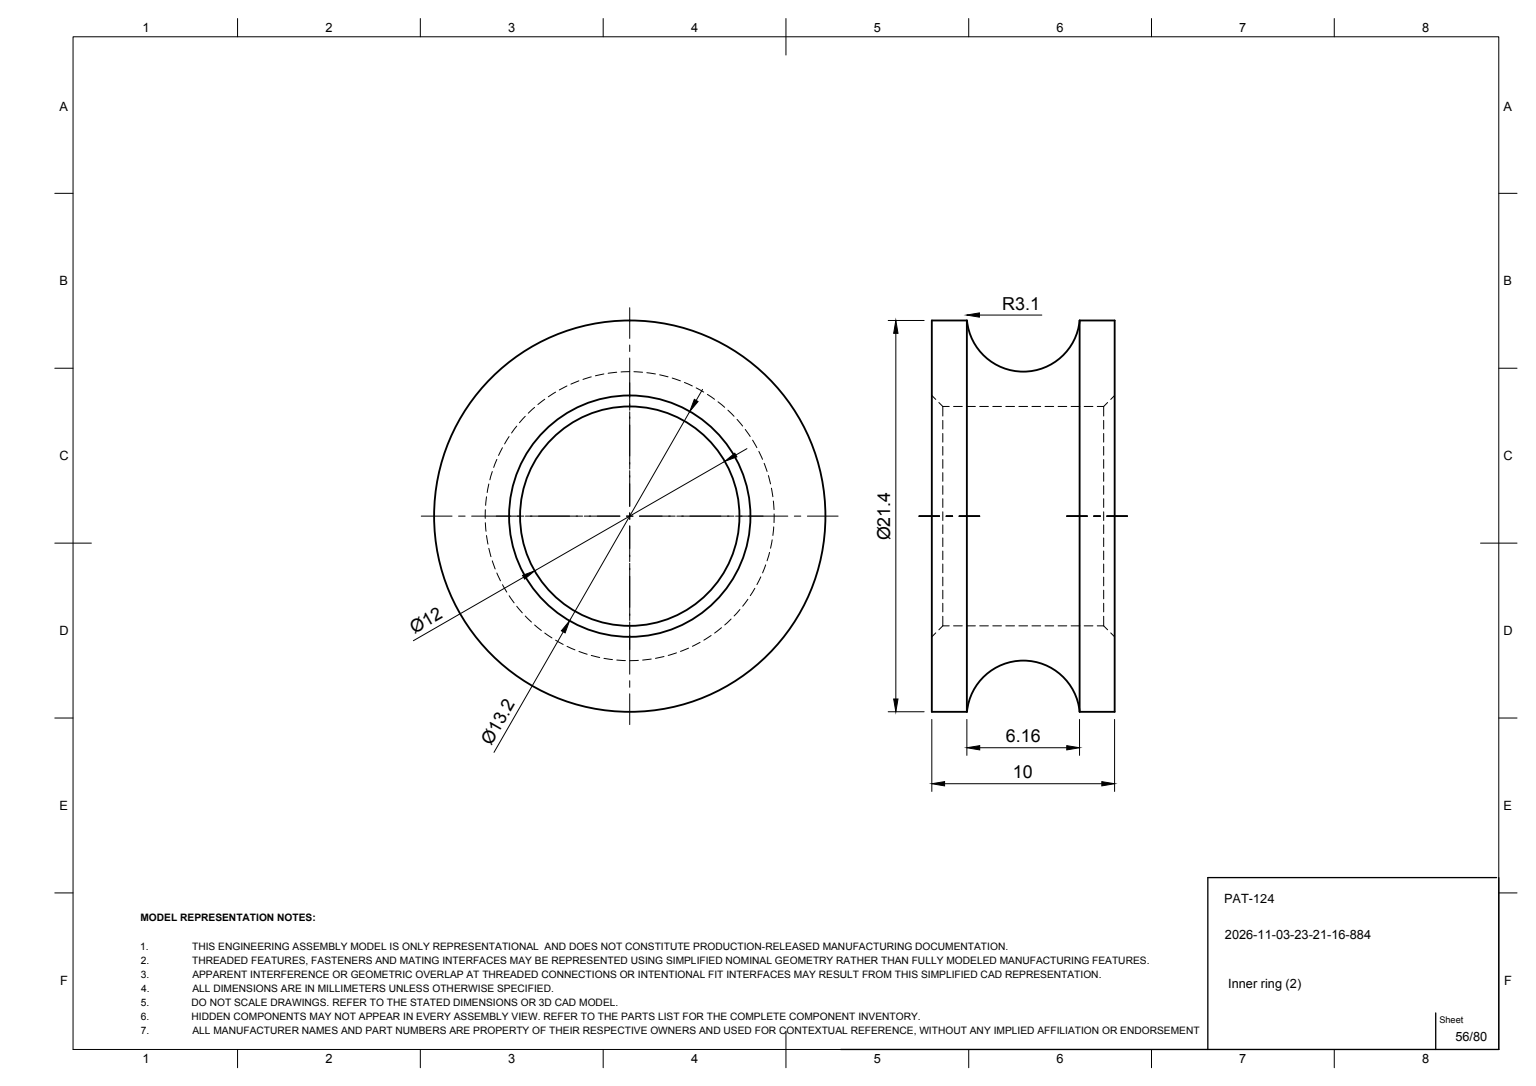
ISO-10303-21;
HEADER;
/* Generated by software containing ST-Developer
 * from STEP Tools, Inc. (www.steptools.com) 
 */

FILE_DESCRIPTION(
/* description */ ('XY cross-slide table'),
/* implementation_level */ '2;1');

FILE_NAME(
/* name */ 'Inner ring (2).step',
/* time_stamp */ '2026-10-28T03:22:46-07:00',
/* author */ (''),
/* organization */ (''),
/* preprocessor_version */ 'ST-DEVELOPER v20.2',
/* originating_system */ 'Autodesk Translation Framework v15.17.0.0',
/* authorisation */ '');

FILE_SCHEMA (('AUTOMOTIVE_DESIGN { 1 0 10303 214 3 1 1 }'));
ENDSEC;

DATA;
#10=MECHANICAL_DESIGN_GEOMETRIC_PRESENTATION_REPRESENTATION('',(#1736),#62984);
#1467=CONICAL_SURFACE('',#25543,0.63,0.785398163397448);
#1468=CONICAL_SURFACE('',#25550,0.63,0.785398163397448);
#1500=TOROIDAL_SURFACE('',#25532,1.1,0.309556);
#1555=SHAPE_REPRESENTATION_RELATIONSHIP('SRR','None',#63411,#1638);
#1638=ADVANCED_BREP_SHAPE_REPRESENTATION('',(#1845),#62948);
#1736=STYLED_ITEM('',(#63912),#1845);
#1845=MANIFOLD_SOLID_BREP('Body1',#23034);
#2201=FACE_BOUND('',#5308,.T.);
#2202=FACE_BOUND('',#5311,.T.);
#2662=PLANE('',#25545);
#2663=PLANE('',#25548);
#3675=FACE_OUTER_BOUND('',#5303,.T.);
#3676=FACE_OUTER_BOUND('',#5304,.T.);
#3677=FACE_OUTER_BOUND('',#5305,.T.);
#3678=FACE_OUTER_BOUND('',#5306,.T.);
#3679=FACE_OUTER_BOUND('',#5307,.T.);
#3680=FACE_OUTER_BOUND('',#5309,.T.);
#3681=FACE_OUTER_BOUND('',#5310,.T.);
#3682=FACE_OUTER_BOUND('',#5312,.T.);
#5303=EDGE_LOOP('',(#18628,#18629,#18630,#18631,#18632,#18633));
#5304=EDGE_LOOP('',(#18634,#18635,#18636,#18637,#18638));
#5305=EDGE_LOOP('',(#18639,#18640,#18641,#18642));
#5306=EDGE_LOOP('',(#18643,#18644,#18645,#18646));
#5307=EDGE_LOOP('',(#18647));
#5308=EDGE_LOOP('',(#18648));
#5309=EDGE_LOOP('',(#18649,#18650,#18651,#18652,#18653));
#5310=EDGE_LOOP('',(#18654));
#5311=EDGE_LOOP('',(#18655));
#5312=EDGE_LOOP('',(#18656,#18657,#18658,#18659));
#6837=LINE('',#48546,#8324);
#6838=LINE('',#48552,#8325);
#6839=LINE('',#48556,#8326);
#6840=LINE('',#48562,#8327);
#6841=LINE('',#48567,#8328);
#8324=VECTOR('',#30470,1.070235);
#8325=VECTOR('',#30477,0.6);
#8326=VECTOR('',#30482,0.63);
#8327=VECTOR('',#30491,1.070235);
#8328=VECTOR('',#30498,0.63);
#9467=CIRCLE('',#25533,1.070235);
#9468=CIRCLE('',#25534,1.070235);
#9469=CIRCLE('',#25535,0.309556);
#9470=CIRCLE('',#25536,1.070235);
#9471=CIRCLE('',#25537,1.070235);
#9472=CIRCLE('',#25539,1.070235);
#9473=CIRCLE('',#25541,0.6);
#9474=CIRCLE('',#25542,0.6);
#9475=CIRCLE('',#25544,0.66);
#9476=CIRCLE('',#25547,1.070235);
#9477=CIRCLE('',#25549,0.66);
#11021=VERTEX_POINT('',#48535);
#11022=VERTEX_POINT('',#48536);
#11023=VERTEX_POINT('',#48539);
#11024=VERTEX_POINT('',#48541);
#11025=VERTEX_POINT('',#48545);
#11026=VERTEX_POINT('',#48549);
#11027=VERTEX_POINT('',#48551);
#11028=VERTEX_POINT('',#48555);
#11029=VERTEX_POINT('',#48560);
#11030=VERTEX_POINT('',#48564);
#13698=EDGE_CURVE('',#11021,#11022,#9467,.T.);
#13699=EDGE_CURVE('',#11022,#11021,#9468,.T.);
#13700=EDGE_CURVE('',#11022,#11023,#9469,.T.);
#13701=EDGE_CURVE('',#11024,#11023,#9470,.T.);
#13702=EDGE_CURVE('',#11023,#11024,#9471,.T.);
#13703=EDGE_CURVE('',#11024,#11025,#6837,.T.);
#13704=EDGE_CURVE('',#11025,#11025,#9472,.T.);
#13705=EDGE_CURVE('',#11026,#11026,#9473,.T.);
#13706=EDGE_CURVE('',#11026,#11027,#6838,.T.);
#13707=EDGE_CURVE('',#11027,#11027,#9474,.T.);
#13708=EDGE_CURVE('',#11027,#11028,#6839,.T.);
#13709=EDGE_CURVE('',#11028,#11028,#9475,.T.);
#13710=EDGE_CURVE('',#11029,#11029,#9476,.T.);
#13711=EDGE_CURVE('',#11029,#11021,#6840,.T.);
#13712=EDGE_CURVE('',#11030,#11030,#9477,.T.);
#13713=EDGE_CURVE('',#11030,#11026,#6841,.T.);
#18628=ORIENTED_EDGE('',*,*,#13698,.F.);
#18629=ORIENTED_EDGE('',*,*,#13699,.F.);
#18630=ORIENTED_EDGE('',*,*,#13700,.T.);
#18631=ORIENTED_EDGE('',*,*,#13701,.F.);
#18632=ORIENTED_EDGE('',*,*,#13702,.F.);
#18633=ORIENTED_EDGE('',*,*,#13700,.F.);
#18634=ORIENTED_EDGE('',*,*,#13701,.T.);
#18635=ORIENTED_EDGE('',*,*,#13702,.T.);
#18636=ORIENTED_EDGE('',*,*,#13703,.T.);
#18637=ORIENTED_EDGE('',*,*,#13704,.T.);
#18638=ORIENTED_EDGE('',*,*,#13703,.F.);
#18639=ORIENTED_EDGE('',*,*,#13705,.T.);
#18640=ORIENTED_EDGE('',*,*,#13706,.T.);
#18641=ORIENTED_EDGE('',*,*,#13707,.F.);
#18642=ORIENTED_EDGE('',*,*,#13706,.F.);
#18643=ORIENTED_EDGE('',*,*,#13707,.T.);
#18644=ORIENTED_EDGE('',*,*,#13708,.T.);
#18645=ORIENTED_EDGE('',*,*,#13709,.F.);
#18646=ORIENTED_EDGE('',*,*,#13708,.F.);
#18647=ORIENTED_EDGE('',*,*,#13704,.F.);
#18648=ORIENTED_EDGE('',*,*,#13709,.T.);
#18649=ORIENTED_EDGE('',*,*,#13710,.F.);
#18650=ORIENTED_EDGE('',*,*,#13711,.T.);
#18651=ORIENTED_EDGE('',*,*,#13698,.T.);
#18652=ORIENTED_EDGE('',*,*,#13699,.T.);
#18653=ORIENTED_EDGE('',*,*,#13711,.F.);
#18654=ORIENTED_EDGE('',*,*,#13710,.T.);
#18655=ORIENTED_EDGE('',*,*,#13712,.F.);
#18656=ORIENTED_EDGE('',*,*,#13712,.T.);
#18657=ORIENTED_EDGE('',*,*,#13713,.T.);
#18658=ORIENTED_EDGE('',*,*,#13705,.F.);
#18659=ORIENTED_EDGE('',*,*,#13713,.F.);
#21416=CYLINDRICAL_SURFACE('',#25538,1.070235);
#21417=CYLINDRICAL_SURFACE('',#25540,0.6);
#21418=CYLINDRICAL_SURFACE('',#25546,1.070235);
#22456=ADVANCED_FACE('',(#3675),#1500,.F.);
#22457=ADVANCED_FACE('',(#3676),#21416,.T.);
#22458=ADVANCED_FACE('',(#3677),#21417,.F.);
#22459=ADVANCED_FACE('',(#3678),#1467,.F.);
#22460=ADVANCED_FACE('',(#3679,#2201),#2662,.T.);
#22461=ADVANCED_FACE('',(#3680),#21418,.T.);
#22462=ADVANCED_FACE('',(#3681,#2202),#2663,.T.);
#22463=ADVANCED_FACE('',(#3682),#1468,.F.);
#23034=CLOSED_SHELL('',(#22456,#22457,#22458,#22459,#22460,#22461,#22462,
#22463));
#25531=AXIS2_PLACEMENT_3D('',#48533,#30454,#30455);
#25532=AXIS2_PLACEMENT_3D('',#48534,#30456,#30457);
#25533=AXIS2_PLACEMENT_3D('',#48537,#30458,#30459);
#25534=AXIS2_PLACEMENT_3D('',#48538,#30460,#30461);
#25535=AXIS2_PLACEMENT_3D('',#48540,#30462,#30463);
#25536=AXIS2_PLACEMENT_3D('',#48542,#30464,#30465);
#25537=AXIS2_PLACEMENT_3D('',#48543,#30466,#30467);
#25538=AXIS2_PLACEMENT_3D('',#48544,#30468,#30469);
#25539=AXIS2_PLACEMENT_3D('',#48547,#30471,#30472);
#25540=AXIS2_PLACEMENT_3D('',#48548,#30473,#30474);
#25541=AXIS2_PLACEMENT_3D('',#48550,#30475,#30476);
#25542=AXIS2_PLACEMENT_3D('',#48553,#30478,#30479);
#25543=AXIS2_PLACEMENT_3D('',#48554,#30480,#30481);
#25544=AXIS2_PLACEMENT_3D('',#48557,#30483,#30484);
#25545=AXIS2_PLACEMENT_3D('',#48558,#30485,#30486);
#25546=AXIS2_PLACEMENT_3D('',#48559,#30487,#30488);
#25547=AXIS2_PLACEMENT_3D('',#48561,#30489,#30490);
#25548=AXIS2_PLACEMENT_3D('',#48563,#30492,#30493);
#25549=AXIS2_PLACEMENT_3D('',#48565,#30494,#30495);
#25550=AXIS2_PLACEMENT_3D('',#48566,#30496,#30497);
#30454=DIRECTION('axis',(0.,0.,1.));
#30455=DIRECTION('refdir',(1.,0.,0.));
#30456=DIRECTION('center_axis',(0.,-1.,0.));
#30457=DIRECTION('ref_axis',(0.,0.,-1.));
#30458=DIRECTION('center_axis',(0.,-1.,0.));
#30459=DIRECTION('ref_axis',(1.,0.,0.));
#30460=DIRECTION('center_axis',(0.,-1.,0.));
#30461=DIRECTION('ref_axis',(1.,0.,0.));
#30462=DIRECTION('center_axis',(1.,0.,1.22464679914735E-16));
#30463=DIRECTION('ref_axis',(-1.22464679914735E-16,0.,1.));
#30464=DIRECTION('center_axis',(0.,1.,0.));
#30465=DIRECTION('ref_axis',(1.,0.,0.));
#30466=DIRECTION('center_axis',(0.,1.,0.));
#30467=DIRECTION('ref_axis',(1.,0.,0.));
#30468=DIRECTION('center_axis',(0.,-1.,0.));
#30469=DIRECTION('ref_axis',(1.,0.,0.));
#30470=DIRECTION('',(0.,1.,0.));
#30471=DIRECTION('center_axis',(0.,-1.,0.));
#30472=DIRECTION('ref_axis',(1.,0.,0.));
#30473=DIRECTION('center_axis',(0.,-1.,0.));
#30474=DIRECTION('ref_axis',(1.,0.,0.));
#30475=DIRECTION('center_axis',(0.,-1.,0.));
#30476=DIRECTION('ref_axis',(1.,0.,0.));
#30477=DIRECTION('',(0.,1.,0.));
#30478=DIRECTION('center_axis',(0.,-1.,0.));
#30479=DIRECTION('ref_axis',(1.,0.,0.));
#30480=DIRECTION('center_axis',(0.,1.,0.));
#30481=DIRECTION('ref_axis',(1.,0.,0.));
#30482=DIRECTION('',(-0.707106781186548,0.707106781186547,-8.65956056235493E-17));
#30483=DIRECTION('center_axis',(0.,-1.,0.));
#30484=DIRECTION('ref_axis',(1.,0.,0.));
#30485=DIRECTION('center_axis',(0.,1.,0.));
#30486=DIRECTION('ref_axis',(0.,0.,1.));
#30487=DIRECTION('center_axis',(0.,-1.,0.));
#30488=DIRECTION('ref_axis',(1.,0.,0.));
#30489=DIRECTION('center_axis',(0.,-1.,0.));
#30490=DIRECTION('ref_axis',(1.,0.,0.));
#30491=DIRECTION('',(0.,1.,0.));
#30492=DIRECTION('center_axis',(0.,-1.,0.));
#30493=DIRECTION('ref_axis',(0.,0.,-1.));
#30494=DIRECTION('center_axis',(0.,-1.,0.));
#30495=DIRECTION('ref_axis',(1.,0.,0.));
#30496=DIRECTION('center_axis',(0.,-1.,0.));
#30497=DIRECTION('ref_axis',(1.,0.,0.));
#30498=DIRECTION('',(0.707106781186548,0.707106781186547,8.65956056235493E-17));
#48533=CARTESIAN_POINT('',(0.,0.,0.));
#48534=CARTESIAN_POINT('Origin',(0.,0.,0.));
#48535=CARTESIAN_POINT('',(-1.070235,-0.308121667383195,-1.31065986708547E-16));
#48536=CARTESIAN_POINT('',(-1.31065986708547E-16,-0.308121667383195,1.070235));
#48537=CARTESIAN_POINT('Origin',(0.,-0.308121667383195,0.));
#48538=CARTESIAN_POINT('Origin',(0.,-0.308121667383195,0.));
#48539=CARTESIAN_POINT('',(-1.31065986708547E-16,0.308121667383195,1.070235));
#48540=CARTESIAN_POINT('Origin',(-1.34711147906209E-16,0.,1.1));
#48541=CARTESIAN_POINT('',(-1.070235,0.308121667383195,1.31065986708547E-16));
#48542=CARTESIAN_POINT('Origin',(0.,0.308121667383195,0.));
#48543=CARTESIAN_POINT('Origin',(0.,0.308121667383195,0.));
#48544=CARTESIAN_POINT('Origin',(0.,0.,0.));
#48545=CARTESIAN_POINT('',(-1.070235,0.5,-1.31065986708547E-16));
#48546=CARTESIAN_POINT('',(-1.070235,0.,-1.31065986708547E-16));
#48547=CARTESIAN_POINT('Origin',(0.,0.5,0.));
#48548=CARTESIAN_POINT('Origin',(0.,0.,0.));
#48549=CARTESIAN_POINT('',(-0.6,-0.44,-7.34788079488412E-17));
#48550=CARTESIAN_POINT('Origin',(0.,-0.44,0.));
#48551=CARTESIAN_POINT('',(-0.6,0.44,-7.34788079488412E-17));
#48552=CARTESIAN_POINT('',(-0.6,0.,-7.34788079488412E-17));
#48553=CARTESIAN_POINT('Origin',(0.,0.44,0.));
#48554=CARTESIAN_POINT('Origin',(0.,0.47,0.));
#48555=CARTESIAN_POINT('',(-0.66,0.5,-8.08266887437253E-17));
#48556=CARTESIAN_POINT('',(-0.63,0.47,-7.71527483462832E-17));
#48557=CARTESIAN_POINT('Origin',(0.,0.5,0.));
#48558=CARTESIAN_POINT('Origin',(1.070235,0.5,0.));
#48559=CARTESIAN_POINT('Origin',(0.,0.,0.));
#48560=CARTESIAN_POINT('',(-1.070235,-0.5,-1.31065986708547E-16));
#48561=CARTESIAN_POINT('Origin',(0.,-0.5,0.));
#48562=CARTESIAN_POINT('',(-1.070235,0.,-1.31065986708547E-16));
#48563=CARTESIAN_POINT('Origin',(0.66,-0.5,0.));
#48564=CARTESIAN_POINT('',(-0.66,-0.5,-8.08266887437253E-17));
#48565=CARTESIAN_POINT('Origin',(0.,-0.5,0.));
#48566=CARTESIAN_POINT('Origin',(0.,-0.47,0.));
#48567=CARTESIAN_POINT('',(-0.63,-0.47,-7.71527483462832E-17));
#62849=UNCERTAINTY_MEASURE_WITH_UNIT(LENGTH_MEASURE(0.001),#62985,
'DISTANCE_ACCURACY_VALUE',
'Maximum model space distance between geometric entities at asserted c
onnectivities');
#62885=UNCERTAINTY_MEASURE_WITH_UNIT(LENGTH_MEASURE(0.001),#62985,
'DISTANCE_ACCURACY_VALUE',
'Maximum model space distance between geometric entities at asserted c
onnectivities');
#62948=(
GEOMETRIC_REPRESENTATION_CONTEXT(3)
GLOBAL_UNCERTAINTY_ASSIGNED_CONTEXT((#62849))
GLOBAL_UNIT_ASSIGNED_CONTEXT((#62985,#62987,#62988))
REPRESENTATION_CONTEXT('','3D')
);
#62984=(
GEOMETRIC_REPRESENTATION_CONTEXT(3)
GLOBAL_UNCERTAINTY_ASSIGNED_CONTEXT((#62885))
GLOBAL_UNIT_ASSIGNED_CONTEXT((#62985,#62987,#62988))
REPRESENTATION_CONTEXT('','3D')
);
#62985=(
LENGTH_UNIT()
NAMED_UNIT(*)
SI_UNIT(.CENTI.,.METRE.)
);
#62987=(
NAMED_UNIT(*)
PLANE_ANGLE_UNIT()
SI_UNIT($,.RADIAN.)
);
#62988=(
NAMED_UNIT(*)
SI_UNIT($,.STERADIAN.)
SOLID_ANGLE_UNIT()
);
#63051=SHAPE_DEFINITION_REPRESENTATION(#63229,#63411);
#63229=PRODUCT_DEFINITION_SHAPE('',$,#63510);
#63411=SHAPE_REPRESENTATION('',(#25531),#62948);
#63447=PRODUCT_DEFINITION_CONTEXT('part definition',#63743,'design');
#63510=PRODUCT_DEFINITION('Inner ring (2)','Inner ring (2)',#63608,#63447);
#63608=PRODUCT_DEFINITION_FORMATION('',$,#63807);
#63743=APPLICATION_CONTEXT(
'Core Data for Automotive Mechanical Design Process');
#63744=PRODUCT_CONTEXT('part definition',#63743,'mechanical');
#63807=PRODUCT('Inner ring (2)','Inner ring (2)','Inner ring (2)',(#63744));
#63906=COLOUR_RGB('Grey',0.48,0.52,0.57);
#63907=FILL_AREA_STYLE_COLOUR('',#63906);
#63908=FILL_AREA_STYLE('',(#63907));
#63909=SURFACE_STYLE_FILL_AREA(#63908);
#63910=SURFACE_SIDE_STYLE('',(#63909));
#63911=SURFACE_STYLE_USAGE(.BOTH.,#63910);
#63912=PRESENTATION_STYLE_ASSIGNMENT((#63911));
ENDSEC;
END-ISO-10303-21;
